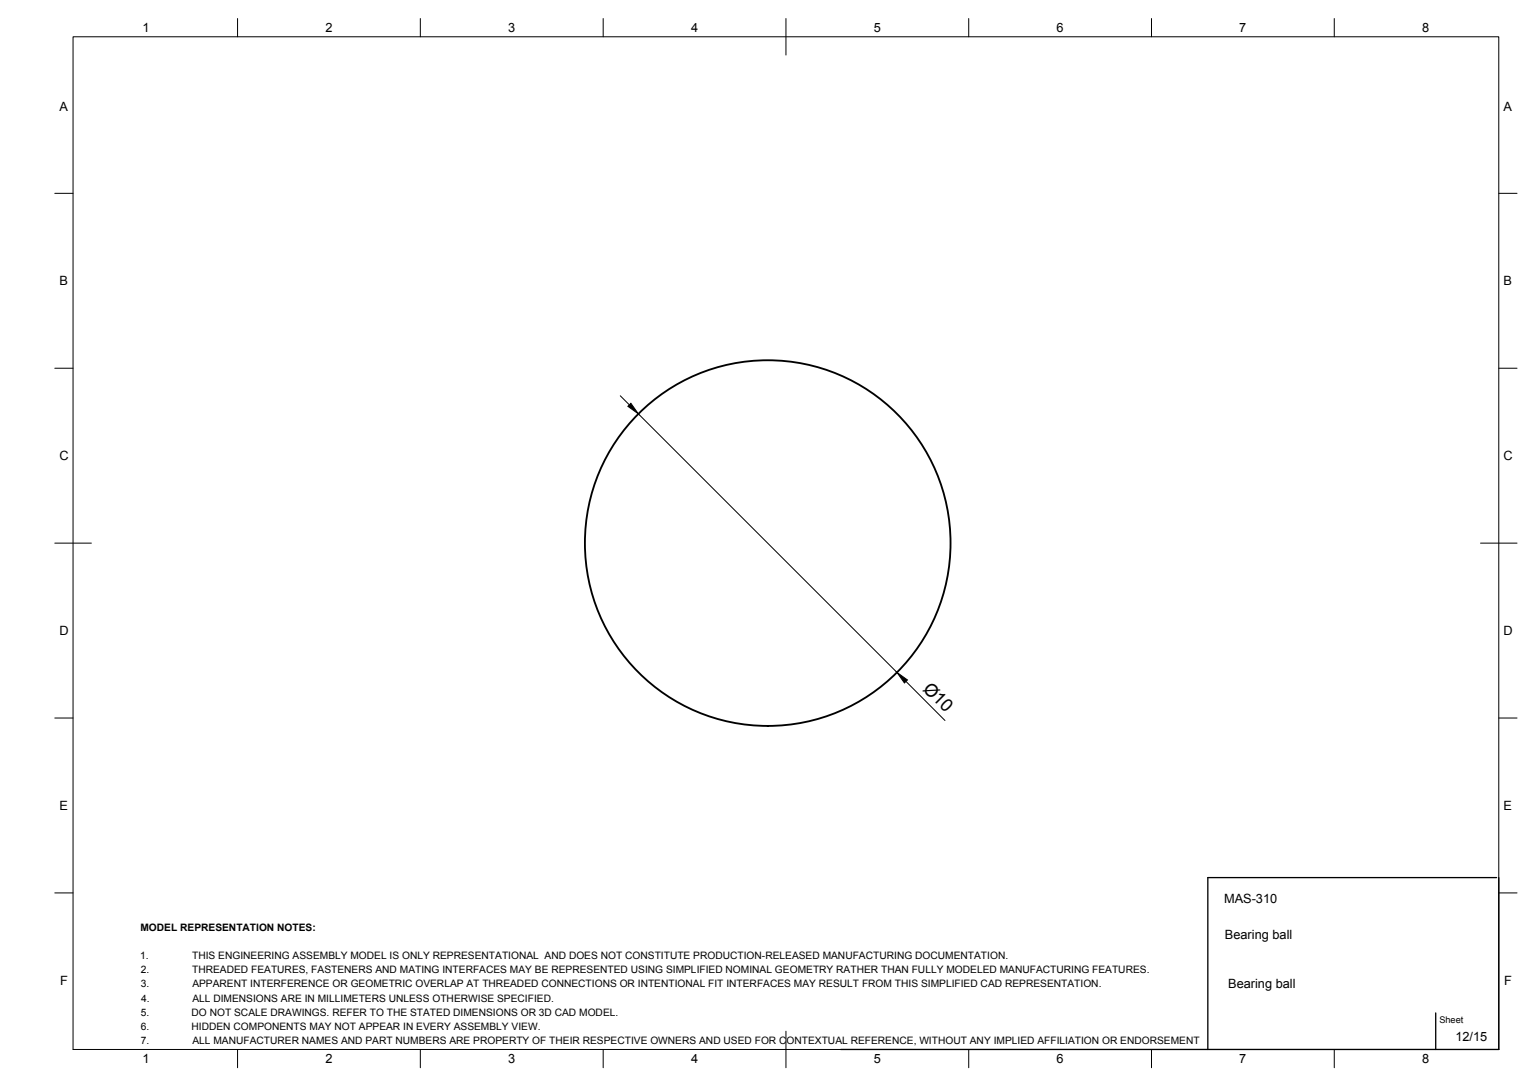
ISO-10303-21;
HEADER;
/* Generated by software containing ST-Developer
 * from STEP Tools, Inc. (www.steptools.com) 
 */

FILE_DESCRIPTION(
/* description */ ('Independent30mm screw-fed quill/spindle unit with16mm straight tool s
ocket, radial set screw, native reusable open ball bearings, retained 
inner/outer race stacks, keyed quill guide and M12x1.75 fine feed. Ext
ernal moving drive and tool not included. Ideal cage orbital links; in
dividual ball spin, force and preload not simulated. No drilling capac
ity, runout, speed, torque, load, life or machine safety rating.'),
/* implementation_level */ '2;1');

FILE_NAME(
/* name */ 'Bearing ball.step',
/* time_stamp */ '2026-11-08T18:59:42-08:00',
/* author */ (''),
/* organization */ (''),
/* preprocessor_version */ 'ST-DEVELOPER v20.2',
/* originating_system */ 'Autodesk Translation Framework v15.17.0.0',
/* authorisation */ '');

FILE_SCHEMA (('AUTOMOTIVE_DESIGN { 1 0 10303 214 3 1 1 }'));
ENDSEC;

DATA;
#10=MECHANICAL_DESIGN_GEOMETRIC_PRESENTATION_REPRESENTATION('',(#1606),#63898);
#223=SPHERICAL_SURFACE('',#16649,5.);
#1570=SHAPE_REPRESENTATION_RELATIONSHIP('SRR','None',#64009,#1588);
#1588=ADVANCED_BREP_SHAPE_REPRESENTATION('',(#1624),#63894);
#1606=STYLED_ITEM('',(#64104),#1624);
#1624=MANIFOLD_SOLID_BREP('Body1',#15492);
#2584=CIRCLE('',#16650,5.);
#3418=FACE_OUTER_BOUND('',#4338,.T.);
#4338=EDGE_LOOP('',(#14030,#14031));
#7342=VERTEX_POINT('',#60427);
#7343=VERTEX_POINT('',#60428);
#9604=EDGE_CURVE('',#7342,#7343,#2584,.T.);
#14030=ORIENTED_EDGE('',*,*,#9604,.T.);
#14031=ORIENTED_EDGE('',*,*,#9604,.F.);
#15398=ADVANCED_FACE('',(#3418),#223,.T.);
#15492=CLOSED_SHELL('',(#15398));
#16648=AXIS2_PLACEMENT_3D('',#60425,#19472,#19473);
#16649=AXIS2_PLACEMENT_3D('',#60426,#19474,#19475);
#16650=AXIS2_PLACEMENT_3D('',#60429,#19476,#19477);
#19472=DIRECTION('axis',(0.,0.,1.));
#19473=DIRECTION('refdir',(1.,0.,0.));
#19474=DIRECTION('center_axis',(6.12323399573677E-17,0.,1.));
#19475=DIRECTION('ref_axis',(1.,0.,0.));
#19476=DIRECTION('center_axis',(1.22464679914735E-16,-1.,0.));
#19477=DIRECTION('ref_axis',(-1.,-1.22464679914735E-16,0.));
#60425=CARTESIAN_POINT('',(0.,0.,0.));
#60426=CARTESIAN_POINT('Origin',(0.,0.,0.));
#60427=CARTESIAN_POINT('',(-3.06161699786838E-16,-3.74939945665464E-32,
5.));
#60428=CARTESIAN_POINT('',(-3.06161699786838E-16,-3.74939945665464E-32,
-5.));
#60429=CARTESIAN_POINT('Origin',(0.,0.,0.));
#63874=UNCERTAINTY_MEASURE_WITH_UNIT(LENGTH_MEASURE(0.01),#63899,
'DISTANCE_ACCURACY_VALUE',
'Maximum model space distance between geometric entities at asserted c
onnectivities');
#63878=UNCERTAINTY_MEASURE_WITH_UNIT(LENGTH_MEASURE(0.01),#63899,
'DISTANCE_ACCURACY_VALUE',
'Maximum model space distance between geometric entities at asserted c
onnectivities');
#63894=(
GEOMETRIC_REPRESENTATION_CONTEXT(3)
GLOBAL_UNCERTAINTY_ASSIGNED_CONTEXT((#63874))
GLOBAL_UNIT_ASSIGNED_CONTEXT((#63899,#63901,#63902))
REPRESENTATION_CONTEXT('','3D')
);
#63898=(
GEOMETRIC_REPRESENTATION_CONTEXT(3)
GLOBAL_UNCERTAINTY_ASSIGNED_CONTEXT((#63878))
GLOBAL_UNIT_ASSIGNED_CONTEXT((#63899,#63901,#63902))
REPRESENTATION_CONTEXT('','3D')
);
#63899=(
LENGTH_UNIT()
NAMED_UNIT(*)
SI_UNIT(.MILLI.,.METRE.)
);
#63901=(
NAMED_UNIT(*)
PLANE_ANGLE_UNIT()
SI_UNIT($,.RADIAN.)
);
#63902=(
NAMED_UNIT(*)
SI_UNIT($,.STERADIAN.)
SOLID_ANGLE_UNIT()
);
#63918=SHAPE_DEFINITION_REPRESENTATION(#63937,#64009);
#63937=PRODUCT_DEFINITION_SHAPE('',$,#64029);
#64009=SHAPE_REPRESENTATION('',(#16648),#63894);
#64013=PRODUCT_DEFINITION_CONTEXT('part definition',#64072,'design');
#64029=PRODUCT_DEFINITION('Bearing ball','Bearing ball',#64048,#64013);
#64048=PRODUCT_DEFINITION_FORMATION('',$,#64089);
#64072=APPLICATION_CONTEXT(
'Core Data for Automotive Mechanical Design Process');
#64073=PRODUCT_CONTEXT('part definition',#64072,'mechanical');
#64089=PRODUCT('Bearing ball','Bearing ball',$,(#64073));
#64104=PRESENTATION_STYLE_ASSIGNMENT((#64117));
#64117=SURFACE_STYLE_USAGE(.BOTH.,#64130);
#64130=SURFACE_SIDE_STYLE('',(#64143));
#64143=SURFACE_STYLE_FILL_AREA(#64156);
#64156=FILL_AREA_STYLE('Ball light gray',(#64169));
#64169=FILL_AREA_STYLE_COLOUR('Ball light gray',#64182);
#64182=COLOUR_RGB('Ball light gray',0.784313725490196,0.815686274509804,
0.854901960784314);
ENDSEC;
END-ISO-10303-21;
